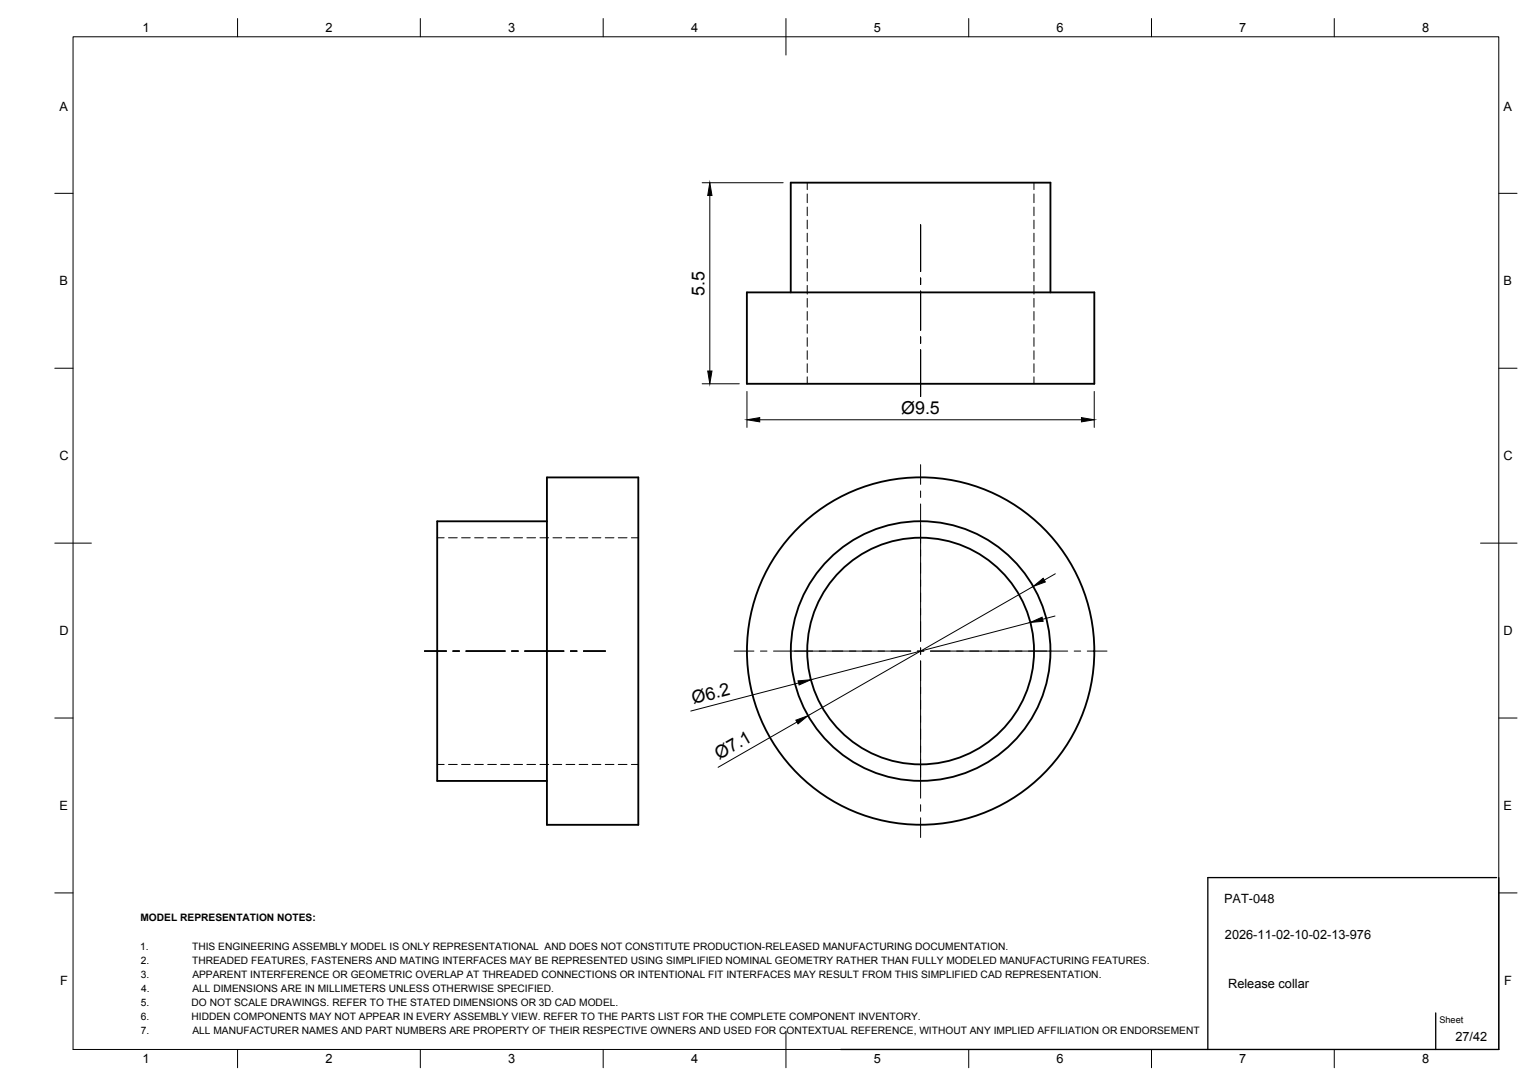
ISO-10303-21;
HEADER;
/* Generated by software containing ST-Developer
 * from STEP Tools, Inc. (www.steptools.com) 
 */

FILE_DESCRIPTION(
/* description */ ('Guided pneumatic stop gate'),
/* implementation_level */ '2;1');

FILE_NAME(
/* name */ 'Release collar.step',
/* time_stamp */ '2026-10-27T21:43:45-07:00',
/* author */ (''),
/* organization */ (''),
/* preprocessor_version */ 'ST-DEVELOPER v20.2',
/* originating_system */ 'Autodesk Translation Framework v15.17.0.0',
/* authorisation */ '');

FILE_SCHEMA (('AUTOMOTIVE_DESIGN { 1 0 10303 214 3 1 1 }'));
ENDSEC;

DATA;
#10=MECHANICAL_DESIGN_GEOMETRIC_PRESENTATION_REPRESENTATION('',(#547),#14392);
#463=SHAPE_REPRESENTATION_RELATIONSHIP('SRR','None',#14598,#505);
#505=ADVANCED_BREP_SHAPE_REPRESENTATION('',(#588),#14360);
#547=STYLED_ITEM('',(#14905),#588);
#588=MANIFOLD_SOLID_BREP('Body1',#7888);
#688=FACE_BOUND('',#1864,.T.);
#689=FACE_BOUND('',#1867,.T.);
#690=FACE_BOUND('',#1870,.T.);
#960=PLANE('',#8753);
#961=PLANE('',#8758);
#962=PLANE('',#8762);
#1315=FACE_OUTER_BOUND('',#1863,.T.);
#1316=FACE_OUTER_BOUND('',#1865,.T.);
#1317=FACE_OUTER_BOUND('',#1866,.T.);
#1318=FACE_OUTER_BOUND('',#1868,.T.);
#1319=FACE_OUTER_BOUND('',#1869,.T.);
#1320=FACE_OUTER_BOUND('',#1871,.T.);
#1863=EDGE_LOOP('',(#6100));
#1864=EDGE_LOOP('',(#6101));
#1865=EDGE_LOOP('',(#6102,#6103,#6104,#6105));
#1866=EDGE_LOOP('',(#6106));
#1867=EDGE_LOOP('',(#6107));
#1868=EDGE_LOOP('',(#6108,#6109,#6110,#6111));
#1869=EDGE_LOOP('',(#6112));
#1870=EDGE_LOOP('',(#6113));
#1871=EDGE_LOOP('',(#6114,#6115,#6116,#6117));
#2514=LINE('',#12781,#3059);
#2515=LINE('',#12788,#3060);
#2516=LINE('',#12793,#3061);
#3059=VECTOR('',#10365,0.475);
#3060=VECTOR('',#10374,0.355);
#3061=VECTOR('',#10381,0.31);
#3510=CIRCLE('',#8754,0.475);
#3511=CIRCLE('',#8755,0.31);
#3512=CIRCLE('',#8757,0.475);
#3513=CIRCLE('',#8759,0.355);
#3514=CIRCLE('',#8761,0.355);
#3515=CIRCLE('',#8763,0.31);
#3985=VERTEX_POINT('',#12774);
#3986=VERTEX_POINT('',#12776);
#3987=VERTEX_POINT('',#12779);
#3988=VERTEX_POINT('',#12783);
#3989=VERTEX_POINT('',#12786);
#3990=VERTEX_POINT('',#12790);
#4748=EDGE_CURVE('',#3985,#3985,#3510,.T.);
#4749=EDGE_CURVE('',#3986,#3986,#3511,.T.);
#4750=EDGE_CURVE('',#3987,#3987,#3512,.T.);
#4751=EDGE_CURVE('',#3987,#3985,#2514,.T.);
#4752=EDGE_CURVE('',#3988,#3988,#3513,.T.);
#4753=EDGE_CURVE('',#3989,#3989,#3514,.T.);
#4754=EDGE_CURVE('',#3989,#3988,#2515,.T.);
#4755=EDGE_CURVE('',#3990,#3990,#3515,.T.);
#4756=EDGE_CURVE('',#3990,#3986,#2516,.T.);
#6100=ORIENTED_EDGE('',*,*,#4748,.F.);
#6101=ORIENTED_EDGE('',*,*,#4749,.T.);
#6102=ORIENTED_EDGE('',*,*,#4750,.F.);
#6103=ORIENTED_EDGE('',*,*,#4751,.T.);
#6104=ORIENTED_EDGE('',*,*,#4748,.T.);
#6105=ORIENTED_EDGE('',*,*,#4751,.F.);
#6106=ORIENTED_EDGE('',*,*,#4750,.T.);
#6107=ORIENTED_EDGE('',*,*,#4752,.F.);
#6108=ORIENTED_EDGE('',*,*,#4753,.F.);
#6109=ORIENTED_EDGE('',*,*,#4754,.T.);
#6110=ORIENTED_EDGE('',*,*,#4752,.T.);
#6111=ORIENTED_EDGE('',*,*,#4754,.F.);
#6112=ORIENTED_EDGE('',*,*,#4753,.T.);
#6113=ORIENTED_EDGE('',*,*,#4755,.F.);
#6114=ORIENTED_EDGE('',*,*,#4755,.T.);
#6115=ORIENTED_EDGE('',*,*,#4756,.T.);
#6116=ORIENTED_EDGE('',*,*,#4749,.F.);
#6117=ORIENTED_EDGE('',*,*,#4756,.F.);
#7304=CYLINDRICAL_SURFACE('',#8756,0.475);
#7305=CYLINDRICAL_SURFACE('',#8760,0.355);
#7306=CYLINDRICAL_SURFACE('',#8764,0.31);
#7597=ADVANCED_FACE('',(#1315,#688),#960,.T.);
#7598=ADVANCED_FACE('',(#1316),#7304,.T.);
#7599=ADVANCED_FACE('',(#1317,#689),#961,.T.);
#7600=ADVANCED_FACE('',(#1318),#7305,.T.);
#7601=ADVANCED_FACE('',(#1319,#690),#962,.T.);
#7602=ADVANCED_FACE('',(#1320),#7306,.F.);
#7888=CLOSED_SHELL('',(#7597,#7598,#7599,#7600,#7601,#7602));
#8752=AXIS2_PLACEMENT_3D('',#12772,#10353,#10354);
#8753=AXIS2_PLACEMENT_3D('',#12773,#10355,#10356);
#8754=AXIS2_PLACEMENT_3D('',#12775,#10357,#10358);
#8755=AXIS2_PLACEMENT_3D('',#12777,#10359,#10360);
#8756=AXIS2_PLACEMENT_3D('',#12778,#10361,#10362);
#8757=AXIS2_PLACEMENT_3D('',#12780,#10363,#10364);
#8758=AXIS2_PLACEMENT_3D('',#12782,#10366,#10367);
#8759=AXIS2_PLACEMENT_3D('',#12784,#10368,#10369);
#8760=AXIS2_PLACEMENT_3D('',#12785,#10370,#10371);
#8761=AXIS2_PLACEMENT_3D('',#12787,#10372,#10373);
#8762=AXIS2_PLACEMENT_3D('',#12789,#10375,#10376);
#8763=AXIS2_PLACEMENT_3D('',#12791,#10377,#10378);
#8764=AXIS2_PLACEMENT_3D('',#12792,#10379,#10380);
#10353=DIRECTION('axis',(0.,0.,1.));
#10354=DIRECTION('refdir',(1.,0.,0.));
#10355=DIRECTION('center_axis',(0.,1.,0.));
#10356=DIRECTION('ref_axis',(0.,0.,1.));
#10357=DIRECTION('center_axis',(0.,-1.,0.));
#10358=DIRECTION('ref_axis',(1.,0.,0.));
#10359=DIRECTION('center_axis',(0.,-1.,0.));
#10360=DIRECTION('ref_axis',(1.,0.,0.));
#10361=DIRECTION('center_axis',(0.,-1.,0.));
#10362=DIRECTION('ref_axis',(1.,0.,0.));
#10363=DIRECTION('center_axis',(0.,-1.,0.));
#10364=DIRECTION('ref_axis',(1.,0.,0.));
#10365=DIRECTION('',(0.,1.,0.));
#10366=DIRECTION('center_axis',(0.,-1.,0.));
#10367=DIRECTION('ref_axis',(0.,0.,-1.));
#10368=DIRECTION('center_axis',(0.,-1.,0.));
#10369=DIRECTION('ref_axis',(1.,0.,0.));
#10370=DIRECTION('center_axis',(0.,-1.,0.));
#10371=DIRECTION('ref_axis',(1.,0.,0.));
#10372=DIRECTION('center_axis',(0.,-1.,0.));
#10373=DIRECTION('ref_axis',(1.,0.,0.));
#10374=DIRECTION('',(0.,1.,0.));
#10375=DIRECTION('center_axis',(0.,-1.,0.));
#10376=DIRECTION('ref_axis',(0.,0.,-1.));
#10377=DIRECTION('center_axis',(0.,-1.,0.));
#10378=DIRECTION('ref_axis',(1.,0.,0.));
#10379=DIRECTION('center_axis',(0.,-1.,0.));
#10380=DIRECTION('ref_axis',(1.,0.,0.));
#10381=DIRECTION('',(0.,1.,0.));
#12772=CARTESIAN_POINT('',(0.,0.,0.));
#12773=CARTESIAN_POINT('Origin',(0.475,1.95,0.));
#12774=CARTESIAN_POINT('',(-0.475,1.95,-5.81707229594993E-17));
#12775=CARTESIAN_POINT('Origin',(0.,1.95,0.));
#12776=CARTESIAN_POINT('',(-0.31,1.95,-3.7964050773568E-17));
#12777=CARTESIAN_POINT('Origin',(0.,1.95,0.));
#12778=CARTESIAN_POINT('Origin',(0.,1.825,0.));
#12779=CARTESIAN_POINT('',(-0.475,1.7,-5.81707229594993E-17));
#12780=CARTESIAN_POINT('Origin',(0.,1.7,0.));
#12781=CARTESIAN_POINT('',(-0.475,1.825,-5.81707229594993E-17));
#12782=CARTESIAN_POINT('Origin',(0.355,1.7,0.));
#12783=CARTESIAN_POINT('',(-0.355,1.7,-4.3474961369731E-17));
#12784=CARTESIAN_POINT('Origin',(0.,1.7,0.));
#12785=CARTESIAN_POINT('Origin',(0.,1.55,0.));
#12786=CARTESIAN_POINT('',(-0.355,1.4,-4.3474961369731E-17));
#12787=CARTESIAN_POINT('Origin',(0.,1.4,0.));
#12788=CARTESIAN_POINT('',(-0.355,1.55,-4.3474961369731E-17));
#12789=CARTESIAN_POINT('Origin',(0.31,1.4,0.));
#12790=CARTESIAN_POINT('',(-0.31,1.4,-3.7964050773568E-17));
#12791=CARTESIAN_POINT('Origin',(0.,1.4,0.));
#12792=CARTESIAN_POINT('Origin',(0.,1.675,0.));
#12793=CARTESIAN_POINT('',(-0.31,1.675,-3.7964050773568E-17));
#14312=UNCERTAINTY_MEASURE_WITH_UNIT(LENGTH_MEASURE(0.001),#14393,
'DISTANCE_ACCURACY_VALUE',
'Maximum model space distance between geometric entities at asserted c
onnectivities');
#14344=UNCERTAINTY_MEASURE_WITH_UNIT(LENGTH_MEASURE(0.001),#14393,
'DISTANCE_ACCURACY_VALUE',
'Maximum model space distance between geometric entities at asserted c
onnectivities');
#14360=(
GEOMETRIC_REPRESENTATION_CONTEXT(3)
GLOBAL_UNCERTAINTY_ASSIGNED_CONTEXT((#14312))
GLOBAL_UNIT_ASSIGNED_CONTEXT((#14393,#14395,#14396))
REPRESENTATION_CONTEXT('','3D')
);
#14392=(
GEOMETRIC_REPRESENTATION_CONTEXT(3)
GLOBAL_UNCERTAINTY_ASSIGNED_CONTEXT((#14344))
GLOBAL_UNIT_ASSIGNED_CONTEXT((#14393,#14395,#14396))
REPRESENTATION_CONTEXT('','3D')
);
#14393=(
LENGTH_UNIT()
NAMED_UNIT(*)
SI_UNIT(.CENTI.,.METRE.)
);
#14395=(
NAMED_UNIT(*)
PLANE_ANGLE_UNIT()
SI_UNIT($,.RADIAN.)
);
#14396=(
NAMED_UNIT(*)
SI_UNIT($,.STERADIAN.)
SOLID_ANGLE_UNIT()
);
#14412=SHAPE_DEFINITION_REPRESENTATION(#14459,#14598);
#14459=PRODUCT_DEFINITION_SHAPE('',$,#14646);
#14598=SHAPE_REPRESENTATION('',(#8752),#14360);
#14630=PRODUCT_DEFINITION_CONTEXT('part definition',#14773,'design');
#14646=PRODUCT_DEFINITION('Release collar','Release collar',#14693,#14630);
#14693=PRODUCT_DEFINITION_FORMATION('',$,#14790);
#14773=APPLICATION_CONTEXT(
'Core Data for Automotive Mechanical Design Process');
#14774=PRODUCT_CONTEXT('part definition',#14773,'mechanical');
#14790=PRODUCT('Release collar','Release collar','Release collar',(#14774));
#14899=COLOUR_RGB('Off White',0.89,0.88,0.83);
#14900=FILL_AREA_STYLE_COLOUR('',#14899);
#14901=FILL_AREA_STYLE('',(#14900));
#14902=SURFACE_STYLE_FILL_AREA(#14901);
#14903=SURFACE_SIDE_STYLE('',(#14902));
#14904=SURFACE_STYLE_USAGE(.BOTH.,#14903);
#14905=PRESENTATION_STYLE_ASSIGNMENT((#14904));
ENDSEC;
END-ISO-10303-21;
